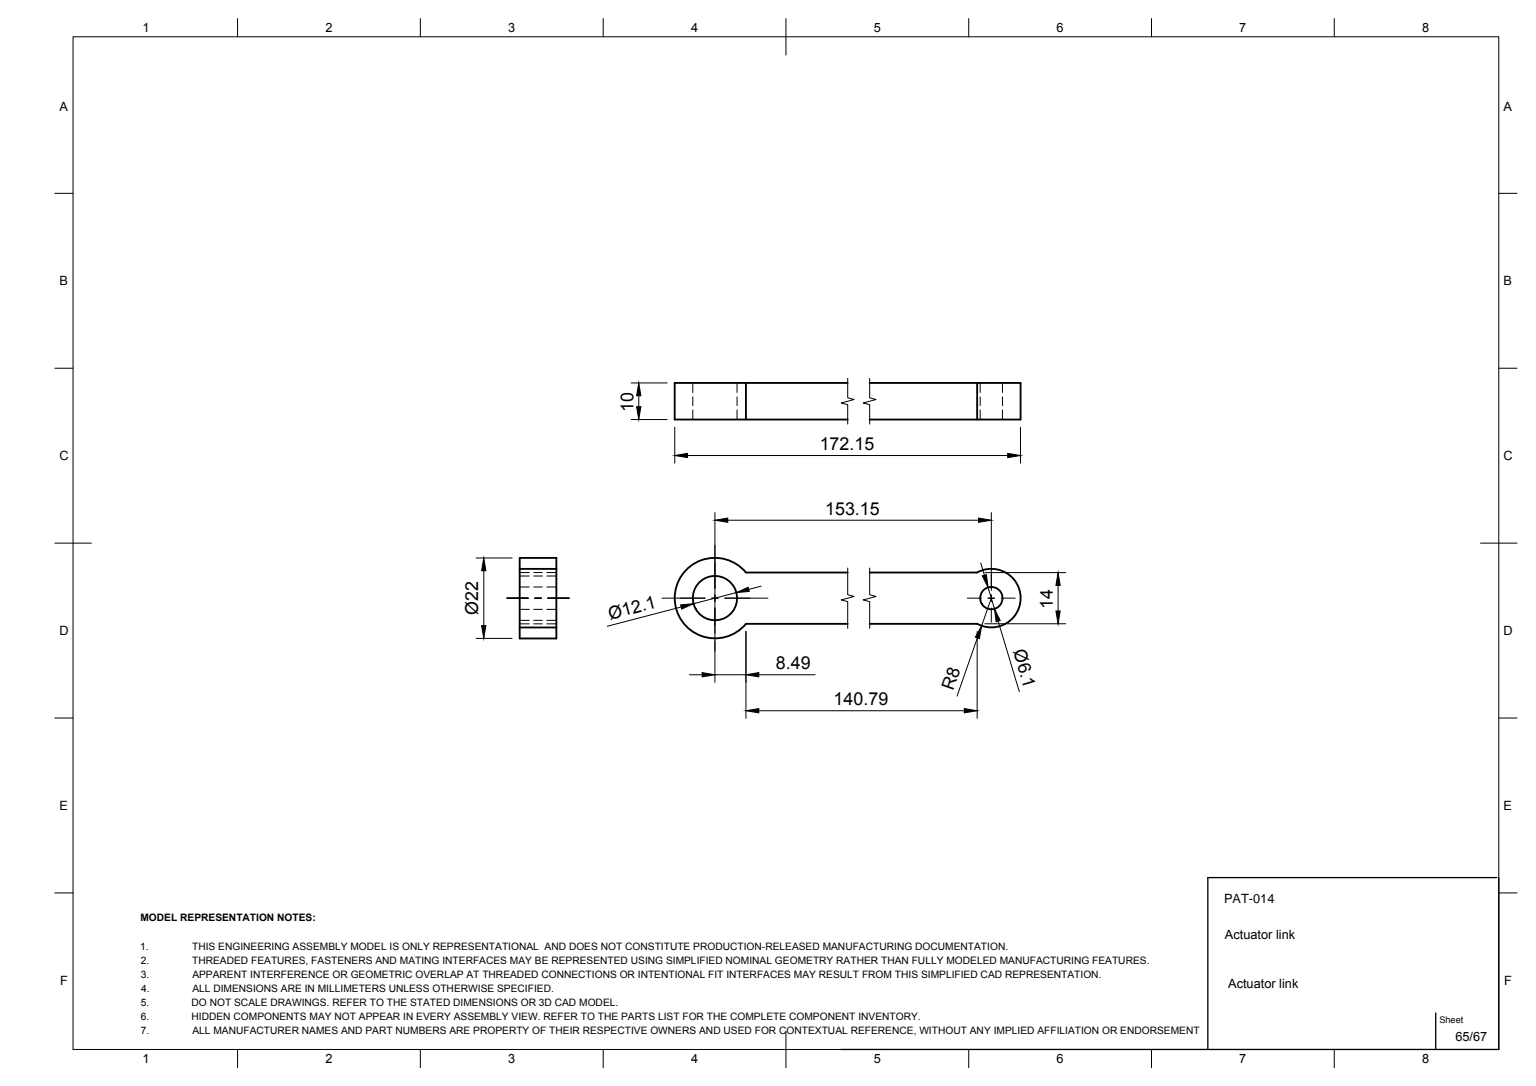
ISO-10303-21;
HEADER;
/* Generated by software containing ST-Developer
 * from STEP Tools, Inc. (www.steptools.com) 
 */

FILE_DESCRIPTION(
/* description */ ('Bin tilter linkage'),
/* implementation_level */ '2;1');

FILE_NAME(
/* name */ 'Actuator link.step',
/* time_stamp */ '2026-10-28T03:26:24-07:00',
/* author */ (''),
/* organization */ (''),
/* preprocessor_version */ 'ST-DEVELOPER v20.2',
/* originating_system */ 'Autodesk Translation Framework v15.17.0.0',
/* authorisation */ '');

FILE_SCHEMA (('AUTOMOTIVE_DESIGN { 1 0 10303 214 3 1 1 }'));
ENDSEC;

DATA;
#10=MECHANICAL_DESIGN_GEOMETRIC_PRESENTATION_REPRESENTATION('',(#970),#23728);
#750=SHAPE_REPRESENTATION_RELATIONSHIP('SRR','None',#24221,#856);
#856=ADVANCED_BREP_SHAPE_REPRESENTATION('',(#1081),#23721);
#970=STYLED_ITEM('',(#24758),#1081);
#1081=MANIFOLD_SOLID_BREP('Body1',#12503);
#1482=FACE_BOUND('',#3816,.T.);
#1483=FACE_BOUND('',#3817,.T.);
#1484=FACE_BOUND('',#3823,.T.);
#1485=FACE_BOUND('',#3824,.T.);
#1876=PLANE('',#15411);
#1877=PLANE('',#15414);
#1878=PLANE('',#15419);
#1879=PLANE('',#15420);
#2641=FACE_OUTER_BOUND('',#3813,.T.);
#2642=FACE_OUTER_BOUND('',#3814,.T.);
#2643=FACE_OUTER_BOUND('',#3815,.T.);
#2644=FACE_OUTER_BOUND('',#3818,.T.);
#2645=FACE_OUTER_BOUND('',#3819,.T.);
#2646=FACE_OUTER_BOUND('',#3820,.T.);
#2647=FACE_OUTER_BOUND('',#3821,.T.);
#2648=FACE_OUTER_BOUND('',#3822,.T.);
#3813=EDGE_LOOP('',(#11183,#11184,#11185,#11186));
#3814=EDGE_LOOP('',(#11187,#11188,#11189,#11190));
#3815=EDGE_LOOP('',(#11191,#11192,#11193,#11194));
#3816=EDGE_LOOP('',(#11195));
#3817=EDGE_LOOP('',(#11196));
#3818=EDGE_LOOP('',(#11197,#11198,#11199,#11200));
#3819=EDGE_LOOP('',(#11201,#11202,#11203,#11204));
#3820=EDGE_LOOP('',(#11205,#11206,#11207,#11208));
#3821=EDGE_LOOP('',(#11209,#11210,#11211,#11212));
#3822=EDGE_LOOP('',(#11213,#11214,#11215,#11216));
#3823=EDGE_LOOP('',(#11217));
#3824=EDGE_LOOP('',(#11218));
#4506=LINE('',#23384,#5181);
#4507=LINE('',#23389,#5182);
#4508=LINE('',#23393,#5183);
#4509=LINE('',#23397,#5184);
#4510=LINE('',#23400,#5185);
#4511=LINE('',#23405,#5186);
#4512=LINE('',#23406,#5187);
#4513=LINE('',#23409,#5188);
#4514=LINE('',#23413,#5189);
#4515=LINE('',#23416,#5190);
#5181=VECTOR('',#19593,0.605);
#5182=VECTOR('',#19598,1.);
#5183=VECTOR('',#19601,1.);
#5184=VECTOR('',#19606,1.);
#5185=VECTOR('',#19609,1.);
#5186=VECTOR('',#19614,1.);
#5187=VECTOR('',#19615,1.);
#5188=VECTOR('',#19618,0.305);
#5189=VECTOR('',#19623,1.);
#5190=VECTOR('',#19628,1.);
#5933=CIRCLE('',#15406,0.605);
#5934=CIRCLE('',#15407,0.605);
#5935=CIRCLE('',#15409,1.1);
#5936=CIRCLE('',#15410,1.1);
#5937=CIRCLE('',#15412,0.8);
#5938=CIRCLE('',#15413,0.305);
#5939=CIRCLE('',#15416,0.305);
#5940=CIRCLE('',#15418,0.8);
#6898=VERTEX_POINT('',#23381);
#6899=VERTEX_POINT('',#23383);
#6900=VERTEX_POINT('',#23387);
#6901=VERTEX_POINT('',#23388);
#6902=VERTEX_POINT('',#23390);
#6903=VERTEX_POINT('',#23392);
#6904=VERTEX_POINT('',#23396);
#6905=VERTEX_POINT('',#23398);
#6906=VERTEX_POINT('',#23401);
#6907=VERTEX_POINT('',#23404);
#6908=VERTEX_POINT('',#23408);
#6909=VERTEX_POINT('',#23412);
#8331=EDGE_CURVE('',#6898,#6898,#5933,.T.);
#8332=EDGE_CURVE('',#6898,#6899,#4506,.T.);
#8333=EDGE_CURVE('',#6899,#6899,#5934,.T.);
#8334=EDGE_CURVE('',#6900,#6901,#4507,.T.);
#8335=EDGE_CURVE('',#6902,#6900,#5935,.T.);
#8336=EDGE_CURVE('',#6903,#6902,#4508,.T.);
#8337=EDGE_CURVE('',#6903,#6901,#5936,.T.);
#8338=EDGE_CURVE('',#6904,#6903,#4509,.T.);
#8339=EDGE_CURVE('',#6905,#6904,#5937,.T.);
#8340=EDGE_CURVE('',#6901,#6905,#4510,.T.);
#8341=EDGE_CURVE('',#6906,#6906,#5938,.T.);
#8342=EDGE_CURVE('',#6907,#6902,#4511,.T.);
#8343=EDGE_CURVE('',#6907,#6904,#4512,.T.);
#8344=EDGE_CURVE('',#6906,#6908,#4513,.T.);
#8345=EDGE_CURVE('',#6908,#6908,#5939,.T.);
#8346=EDGE_CURVE('',#6905,#6909,#4514,.T.);
#8347=EDGE_CURVE('',#6909,#6907,#5940,.T.);
#8348=EDGE_CURVE('',#6900,#6909,#4515,.T.);
#11183=ORIENTED_EDGE('',*,*,#8331,.F.);
#11184=ORIENTED_EDGE('',*,*,#8332,.T.);
#11185=ORIENTED_EDGE('',*,*,#8333,.F.);
#11186=ORIENTED_EDGE('',*,*,#8332,.F.);
#11187=ORIENTED_EDGE('',*,*,#8334,.F.);
#11188=ORIENTED_EDGE('',*,*,#8335,.F.);
#11189=ORIENTED_EDGE('',*,*,#8336,.F.);
#11190=ORIENTED_EDGE('',*,*,#8337,.T.);
#11191=ORIENTED_EDGE('',*,*,#8337,.F.);
#11192=ORIENTED_EDGE('',*,*,#8338,.F.);
#11193=ORIENTED_EDGE('',*,*,#8339,.F.);
#11194=ORIENTED_EDGE('',*,*,#8340,.F.);
#11195=ORIENTED_EDGE('',*,*,#8331,.T.);
#11196=ORIENTED_EDGE('',*,*,#8341,.T.);
#11197=ORIENTED_EDGE('',*,*,#8336,.T.);
#11198=ORIENTED_EDGE('',*,*,#8342,.F.);
#11199=ORIENTED_EDGE('',*,*,#8343,.T.);
#11200=ORIENTED_EDGE('',*,*,#8338,.T.);
#11201=ORIENTED_EDGE('',*,*,#8341,.F.);
#11202=ORIENTED_EDGE('',*,*,#8344,.T.);
#11203=ORIENTED_EDGE('',*,*,#8345,.F.);
#11204=ORIENTED_EDGE('',*,*,#8344,.F.);
#11205=ORIENTED_EDGE('',*,*,#8346,.F.);
#11206=ORIENTED_EDGE('',*,*,#8339,.T.);
#11207=ORIENTED_EDGE('',*,*,#8343,.F.);
#11208=ORIENTED_EDGE('',*,*,#8347,.F.);
#11209=ORIENTED_EDGE('',*,*,#8334,.T.);
#11210=ORIENTED_EDGE('',*,*,#8340,.T.);
#11211=ORIENTED_EDGE('',*,*,#8346,.T.);
#11212=ORIENTED_EDGE('',*,*,#8348,.F.);
#11213=ORIENTED_EDGE('',*,*,#8348,.T.);
#11214=ORIENTED_EDGE('',*,*,#8347,.T.);
#11215=ORIENTED_EDGE('',*,*,#8342,.T.);
#11216=ORIENTED_EDGE('',*,*,#8335,.T.);
#11217=ORIENTED_EDGE('',*,*,#8333,.T.);
#11218=ORIENTED_EDGE('',*,*,#8345,.T.);
#11603=CYLINDRICAL_SURFACE('',#15405,0.605);
#11604=CYLINDRICAL_SURFACE('',#15408,1.1);
#11605=CYLINDRICAL_SURFACE('',#15415,0.305);
#11606=CYLINDRICAL_SURFACE('',#15417,0.8);
#12366=ADVANCED_FACE('',(#2641),#11603,.F.);
#12367=ADVANCED_FACE('',(#2642),#11604,.T.);
#12368=ADVANCED_FACE('',(#2643,#1482,#1483),#1876,.F.);
#12369=ADVANCED_FACE('',(#2644),#1877,.T.);
#12370=ADVANCED_FACE('',(#2645),#11605,.F.);
#12371=ADVANCED_FACE('',(#2646),#11606,.T.);
#12372=ADVANCED_FACE('',(#2647),#1878,.T.);
#12373=ADVANCED_FACE('',(#2648,#1484,#1485),#1879,.T.);
#12503=CLOSED_SHELL('',(#12366,#12367,#12368,#12369,#12370,#12371,#12372,
#12373));
#15404=AXIS2_PLACEMENT_3D('',#23379,#19587,#19588);
#15405=AXIS2_PLACEMENT_3D('',#23380,#19589,#19590);
#15406=AXIS2_PLACEMENT_3D('',#23382,#19591,#19592);
#15407=AXIS2_PLACEMENT_3D('',#23385,#19594,#19595);
#15408=AXIS2_PLACEMENT_3D('',#23386,#19596,#19597);
#15409=AXIS2_PLACEMENT_3D('',#23391,#19599,#19600);
#15410=AXIS2_PLACEMENT_3D('',#23394,#19602,#19603);
#15411=AXIS2_PLACEMENT_3D('',#23395,#19604,#19605);
#15412=AXIS2_PLACEMENT_3D('',#23399,#19607,#19608);
#15413=AXIS2_PLACEMENT_3D('',#23402,#19610,#19611);
#15414=AXIS2_PLACEMENT_3D('',#23403,#19612,#19613);
#15415=AXIS2_PLACEMENT_3D('',#23407,#19616,#19617);
#15416=AXIS2_PLACEMENT_3D('',#23410,#19619,#19620);
#15417=AXIS2_PLACEMENT_3D('',#23411,#19621,#19622);
#15418=AXIS2_PLACEMENT_3D('',#23414,#19624,#19625);
#15419=AXIS2_PLACEMENT_3D('',#23415,#19626,#19627);
#15420=AXIS2_PLACEMENT_3D('',#23417,#19629,#19630);
#19587=DIRECTION('axis',(0.,0.,1.));
#19588=DIRECTION('refdir',(1.,0.,0.));
#19589=DIRECTION('center_axis',(0.,1.,0.));
#19590=DIRECTION('ref_axis',(1.,0.,0.));
#19591=DIRECTION('center_axis',(0.,1.,0.));
#19592=DIRECTION('ref_axis',(1.,0.,0.));
#19593=DIRECTION('',(0.,1.,0.));
#19594=DIRECTION('center_axis',(0.,-1.,0.));
#19595=DIRECTION('ref_axis',(1.,0.,0.));
#19596=DIRECTION('center_axis',(0.,1.,0.));
#19597=DIRECTION('ref_axis',(1.,0.,0.));
#19598=DIRECTION('',(0.,-1.,0.));
#19599=DIRECTION('center_axis',(0.,1.,0.));
#19600=DIRECTION('ref_axis',(1.,0.,0.));
#19601=DIRECTION('',(0.,1.,0.));
#19602=DIRECTION('center_axis',(0.,1.,0.));
#19603=DIRECTION('ref_axis',(1.,0.,0.));
#19604=DIRECTION('center_axis',(0.,1.,0.));
#19605=DIRECTION('ref_axis',(1.,0.,0.));
#19606=DIRECTION('',(0.874781243901175,0.,0.484518085646669));
#19607=DIRECTION('center_axis',(0.,1.,0.));
#19608=DIRECTION('ref_axis',(1.,0.,0.));
#19609=DIRECTION('',(-0.874781243901175,0.,-0.484518085646669));
#19610=DIRECTION('center_axis',(0.,1.,0.));
#19611=DIRECTION('ref_axis',(1.,0.,0.));
#19612=DIRECTION('center_axis',(-0.484518085646669,0.,0.874781243901175));
#19613=DIRECTION('ref_axis',(0.874781243901175,0.,0.484518085646669));
#19614=DIRECTION('',(0.874781243901175,0.,0.484518085646669));
#19615=DIRECTION('',(0.,-1.,0.));
#19616=DIRECTION('center_axis',(0.,1.,0.));
#19617=DIRECTION('ref_axis',(1.,0.,0.));
#19618=DIRECTION('',(0.,1.,0.));
#19619=DIRECTION('center_axis',(0.,-1.,0.));
#19620=DIRECTION('ref_axis',(1.,0.,0.));
#19621=DIRECTION('center_axis',(0.,1.,0.));
#19622=DIRECTION('ref_axis',(-0.874781243901175,0.,-0.48451808564667));
#19623=DIRECTION('',(0.,1.,0.));
#19624=DIRECTION('center_axis',(0.,1.,0.));
#19625=DIRECTION('ref_axis',(1.,0.,0.));
#19626=DIRECTION('center_axis',(0.484518085646669,0.,-0.874781243901175));
#19627=DIRECTION('ref_axis',(-0.874781243901175,0.,-0.484518085646669));
#19628=DIRECTION('',(-0.874781243901175,0.,-0.484518085646669));
#19629=DIRECTION('center_axis',(0.,1.,0.));
#19630=DIRECTION('ref_axis',(0.,0.,1.));
#23379=CARTESIAN_POINT('',(0.,0.,0.));
#23380=CARTESIAN_POINT('Origin',(9.39692620785909,-5.1,18.4202014332567));
#23381=CARTESIAN_POINT('',(8.79192620785908,-5.,18.4202014332567));
#23382=CARTESIAN_POINT('Origin',(9.39692620785909,-5.,18.4202014332567));
#23383=CARTESIAN_POINT('',(8.79192620785908,-4.,18.4202014332567));
#23384=CARTESIAN_POINT('',(8.79192620785908,-5.1,18.4202014332567));
#23385=CARTESIAN_POINT('Origin',(9.39692620785909,-4.,18.4202014332567));
#23386=CARTESIAN_POINT('Origin',(9.39692620785909,-5.,18.4202014332567));
#23387=CARTESIAN_POINT('',(8.99381236827096,-4.,17.3967273337639));
#23388=CARTESIAN_POINT('',(8.99381236827096,-5.,17.3967273337639));
#23389=CARTESIAN_POINT('',(8.99381236827096,-5.,17.3967273337639));
#23390=CARTESIAN_POINT('',(8.31548704836563,-4.,18.6214210752256));
#23391=CARTESIAN_POINT('Origin',(9.39692620785909,-4.,18.4202014332567));
#23392=CARTESIAN_POINT('',(8.31548704836563,-5.,18.6214210752256));
#23393=CARTESIAN_POINT('',(8.31548704836563,-5.,18.6214210752256));
#23394=CARTESIAN_POINT('Origin',(9.39692620785909,-5.,18.4202014332567));
#23395=CARTESIAN_POINT('Origin',(2.69846310392954,-5.,14.7101007166283));
#23396=CARTESIAN_POINT('',(-4.00036134103228,-5.,11.7999999183954));
#23397=CARTESIAN_POINT('',(-4.33916265995267,-5.,11.6123468707308));
#23398=CARTESIAN_POINT('',(-3.32203602112695,-5.,10.5753061769338));
#23399=CARTESIAN_POINT('Origin',(-4.,-5.,11.));
#23400=CARTESIAN_POINT('',(9.73608886781175,-5.,17.8078545625259));
#23401=CARTESIAN_POINT('',(-4.305,-5.,11.));
#23402=CARTESIAN_POINT('Origin',(-4.,-5.,11.));
#23403=CARTESIAN_POINT('Origin',(-4.33916265995267,-5.,11.6123468707308));
#23404=CARTESIAN_POINT('',(-4.00036134103228,-4.,11.7999999183954));
#23405=CARTESIAN_POINT('',(-4.33916265995267,-4.,11.6123468707308));
#23406=CARTESIAN_POINT('',(-4.00036134103228,-5.,11.7999999183954));
#23407=CARTESIAN_POINT('Origin',(-4.,-5.1,11.));
#23408=CARTESIAN_POINT('',(-4.305,-4.,11.));
#23409=CARTESIAN_POINT('',(-4.305,-5.1,11.));
#23410=CARTESIAN_POINT('Origin',(-4.,-4.,11.));
#23411=CARTESIAN_POINT('Origin',(-4.,-5.,11.));
#23412=CARTESIAN_POINT('',(-3.32203602112695,-4.,10.5753061769338));
#23413=CARTESIAN_POINT('',(-3.32203602112695,-5.,10.5753061769338));
#23414=CARTESIAN_POINT('Origin',(-4.,-4.,11.));
#23415=CARTESIAN_POINT('Origin',(9.73608886781175,-5.,17.8078545625259));
#23416=CARTESIAN_POINT('',(9.73608886781175,-4.,17.8078545625259));
#23417=CARTESIAN_POINT('Origin',(2.69846310392954,-4.,14.7101007166283));
#23604=UNCERTAINTY_MEASURE_WITH_UNIT(LENGTH_MEASURE(0.001),#23729,
'DISTANCE_ACCURACY_VALUE',
'Maximum model space distance between geometric entities at asserted c
onnectivities');
#23611=UNCERTAINTY_MEASURE_WITH_UNIT(LENGTH_MEASURE(0.001),#23729,
'DISTANCE_ACCURACY_VALUE',
'Maximum model space distance between geometric entities at asserted c
onnectivities');
#23721=(
GEOMETRIC_REPRESENTATION_CONTEXT(3)
GLOBAL_UNCERTAINTY_ASSIGNED_CONTEXT((#23604))
GLOBAL_UNIT_ASSIGNED_CONTEXT((#23729,#23731,#23732))
REPRESENTATION_CONTEXT('','3D')
);
#23728=(
GEOMETRIC_REPRESENTATION_CONTEXT(3)
GLOBAL_UNCERTAINTY_ASSIGNED_CONTEXT((#23611))
GLOBAL_UNIT_ASSIGNED_CONTEXT((#23729,#23731,#23732))
REPRESENTATION_CONTEXT('','3D')
);
#23729=(
LENGTH_UNIT()
NAMED_UNIT(*)
SI_UNIT(.CENTI.,.METRE.)
);
#23731=(
NAMED_UNIT(*)
PLANE_ANGLE_UNIT()
SI_UNIT($,.RADIAN.)
);
#23732=(
NAMED_UNIT(*)
SI_UNIT($,.STERADIAN.)
SOLID_ANGLE_UNIT()
);
#23842=SHAPE_DEFINITION_REPRESENTATION(#24092,#24221);
#24092=PRODUCT_DEFINITION_SHAPE('',$,#24338);
#24221=SHAPE_REPRESENTATION('',(#15404),#23721);
#24228=PRODUCT_DEFINITION_CONTEXT('part definition',#24578,'design');
#24338=PRODUCT_DEFINITION('Actuator link','Actuator link',#24454,#24228);
#24454=PRODUCT_DEFINITION_FORMATION('',$,#24689);
#24578=APPLICATION_CONTEXT(
'Core Data for Automotive Mechanical Design Process');
#24579=PRODUCT_CONTEXT('part definition',#24578,'mechanical');
#24689=PRODUCT('Actuator link','Actuator link','Actuator link',(#24579));
#24752=COLOUR_RGB('Sky Blue',0.24,0.69,0.87);
#24753=FILL_AREA_STYLE_COLOUR('',#24752);
#24754=FILL_AREA_STYLE('',(#24753));
#24755=SURFACE_STYLE_FILL_AREA(#24754);
#24756=SURFACE_SIDE_STYLE('',(#24755));
#24757=SURFACE_STYLE_USAGE(.BOTH.,#24756);
#24758=PRESENTATION_STYLE_ASSIGNMENT((#24757));
ENDSEC;
END-ISO-10303-21;
